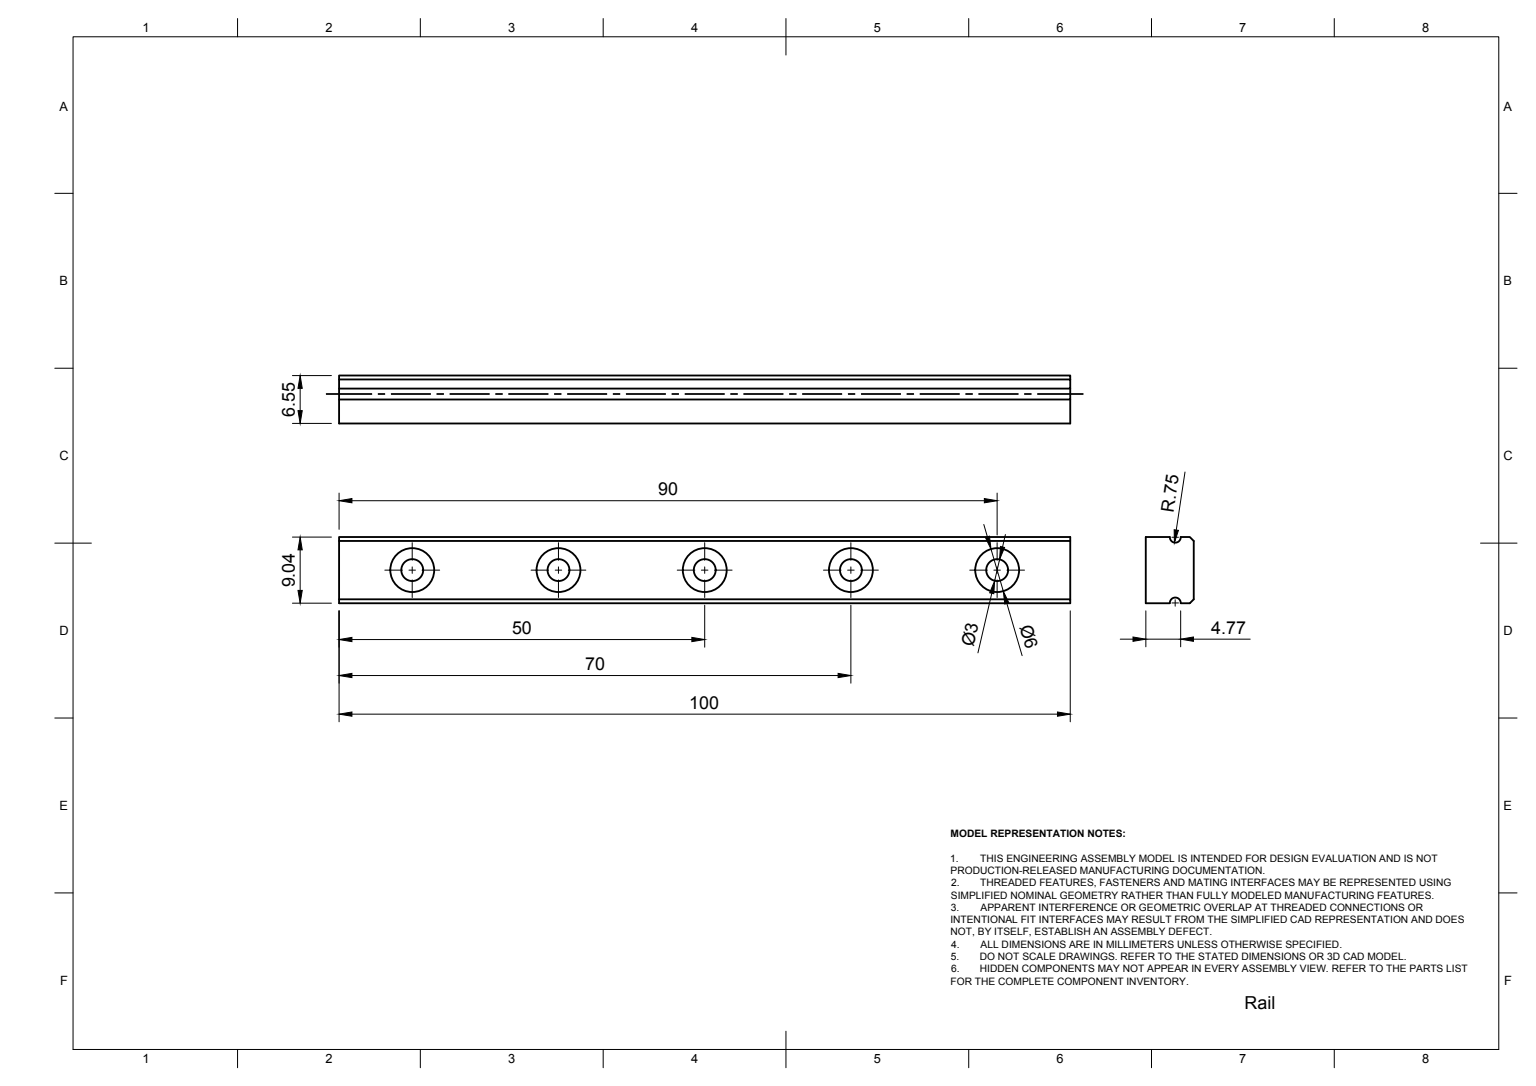
ISO-10303-21;
HEADER;
/* Generated by software containing ST-Developer
 * from STEP Tools, Inc. (www.steptools.com) 
 */

FILE_DESCRIPTION(
/* description */ (''),
/* implementation_level */ '2;1');

FILE_NAME(
/* name */ 'Rail.step',
/* time_stamp */ '2026-10-06T13:23:02-07:00',
/* author */ (''),
/* organization */ (''),
/* preprocessor_version */ 'ST-DEVELOPER v20.2',
/* originating_system */ 'Autodesk Translation Framework v15.15.0.0',
/* authorisation */ '');

FILE_SCHEMA (('AUTOMOTIVE_DESIGN { 1 0 10303 214 3 1 1 }'));
ENDSEC;

DATA;
#10=MECHANICAL_DESIGN_GEOMETRIC_PRESENTATION_REPRESENTATION('',(#75),#4994);
#55=SHAPE_REPRESENTATION_RELATIONSHIP('SRR','None',#5036,#65);
#65=ADVANCED_BREP_SHAPE_REPRESENTATION('',(#85),#4988);
#75=STYLED_ITEM('',(#5092),#85);
#85=MANIFOLD_SOLID_BREP('Body1',#2915);
#99=CYLINDRICAL_SURFACE('',#3150,1.5);
#100=CYLINDRICAL_SURFACE('',#3154,1.5);
#101=CYLINDRICAL_SURFACE('',#3158,1.5);
#102=CYLINDRICAL_SURFACE('',#3162,1.5);
#103=CYLINDRICAL_SURFACE('',#3166,1.5);
#104=CYLINDRICAL_SURFACE('',#3168,3.);
#105=CYLINDRICAL_SURFACE('',#3172,3.);
#106=CYLINDRICAL_SURFACE('',#3176,3.);
#107=CYLINDRICAL_SURFACE('',#3180,3.);
#108=CYLINDRICAL_SURFACE('',#3184,3.);
#109=CYLINDRICAL_SURFACE('',#3189,0.747295203682);
#110=CYLINDRICAL_SURFACE('',#3197,0.747295203682);
#131=FACE_BOUND('',#567,.T.);
#132=FACE_BOUND('',#568,.T.);
#133=FACE_BOUND('',#569,.T.);
#134=FACE_BOUND('',#570,.T.);
#135=FACE_BOUND('',#571,.T.);
#136=FACE_BOUND('',#583,.T.);
#137=FACE_BOUND('',#586,.T.);
#138=FACE_BOUND('',#589,.T.);
#139=FACE_BOUND('',#592,.T.);
#140=FACE_BOUND('',#595,.T.);
#141=FACE_BOUND('',#605,.T.);
#142=FACE_BOUND('',#606,.T.);
#143=FACE_BOUND('',#607,.T.);
#144=FACE_BOUND('',#608,.T.);
#145=FACE_BOUND('',#609,.T.);
#226=PLANE('',#3145);
#227=PLANE('',#3171);
#228=PLANE('',#3175);
#229=PLANE('',#3179);
#230=PLANE('',#3183);
#231=PLANE('',#3187);
#232=PLANE('',#3188);
#233=PLANE('',#3192);
#234=PLANE('',#3193);
#235=PLANE('',#3194);
#236=PLANE('',#3196);
#237=PLANE('',#3199);
#238=PLANE('',#3200);
#239=PLANE('',#3201);
#240=PLANE('',#3202);
#379=FACE_OUTER_BOUND('',#565,.T.);
#380=FACE_OUTER_BOUND('',#566,.T.);
#381=FACE_OUTER_BOUND('',#572,.T.);
#382=FACE_OUTER_BOUND('',#573,.T.);
#383=FACE_OUTER_BOUND('',#574,.T.);
#384=FACE_OUTER_BOUND('',#575,.T.);
#385=FACE_OUTER_BOUND('',#576,.T.);
#386=FACE_OUTER_BOUND('',#577,.T.);
#387=FACE_OUTER_BOUND('',#578,.T.);
#388=FACE_OUTER_BOUND('',#579,.T.);
#389=FACE_OUTER_BOUND('',#580,.T.);
#390=FACE_OUTER_BOUND('',#581,.T.);
#391=FACE_OUTER_BOUND('',#582,.T.);
#392=FACE_OUTER_BOUND('',#584,.T.);
#393=FACE_OUTER_BOUND('',#585,.T.);
#394=FACE_OUTER_BOUND('',#587,.T.);
#395=FACE_OUTER_BOUND('',#588,.T.);
#396=FACE_OUTER_BOUND('',#590,.T.);
#397=FACE_OUTER_BOUND('',#591,.T.);
#398=FACE_OUTER_BOUND('',#593,.T.);
#399=FACE_OUTER_BOUND('',#594,.T.);
#400=FACE_OUTER_BOUND('',#596,.T.);
#401=FACE_OUTER_BOUND('',#597,.T.);
#402=FACE_OUTER_BOUND('',#598,.T.);
#403=FACE_OUTER_BOUND('',#599,.T.);
#404=FACE_OUTER_BOUND('',#600,.T.);
#405=FACE_OUTER_BOUND('',#601,.T.);
#406=FACE_OUTER_BOUND('',#602,.T.);
#407=FACE_OUTER_BOUND('',#603,.T.);
#408=FACE_OUTER_BOUND('',#604,.T.);
#409=FACE_OUTER_BOUND('',#610,.T.);
#410=FACE_OUTER_BOUND('',#611,.T.);
#565=EDGE_LOOP('',(#2248,#2249,#2250,#2251));
#566=EDGE_LOOP('',(#2252,#2253,#2254,#2255));
#567=EDGE_LOOP('',(#2256));
#568=EDGE_LOOP('',(#2257));
#569=EDGE_LOOP('',(#2258));
#570=EDGE_LOOP('',(#2259));
#571=EDGE_LOOP('',(#2260));
#572=EDGE_LOOP('',(#2261,#2262,#2263,#2264));
#573=EDGE_LOOP('',(#2265,#2266,#2267,#2268));
#574=EDGE_LOOP('',(#2269,#2270,#2271,#2272));
#575=EDGE_LOOP('',(#2273,#2274,#2275,#2276));
#576=EDGE_LOOP('',(#2277,#2278,#2279,#2280));
#577=EDGE_LOOP('',(#2281,#2282,#2283,#2284));
#578=EDGE_LOOP('',(#2285,#2286,#2287,#2288));
#579=EDGE_LOOP('',(#2289,#2290,#2291,#2292));
#580=EDGE_LOOP('',(#2293,#2294,#2295,#2296));
#581=EDGE_LOOP('',(#2297,#2298,#2299,#2300));
#582=EDGE_LOOP('',(#2301));
#583=EDGE_LOOP('',(#2302));
#584=EDGE_LOOP('',(#2303,#2304,#2305,#2306));
#585=EDGE_LOOP('',(#2307));
#586=EDGE_LOOP('',(#2308));
#587=EDGE_LOOP('',(#2309,#2310,#2311,#2312));
#588=EDGE_LOOP('',(#2313));
#589=EDGE_LOOP('',(#2314));
#590=EDGE_LOOP('',(#2315,#2316,#2317,#2318));
#591=EDGE_LOOP('',(#2319));
#592=EDGE_LOOP('',(#2320));
#593=EDGE_LOOP('',(#2321,#2322,#2323,#2324));
#594=EDGE_LOOP('',(#2325));
#595=EDGE_LOOP('',(#2326));
#596=EDGE_LOOP('',(#2327,#2328,#2329,#2330));
#597=EDGE_LOOP('',(#2331,#2332,#2333,#2334));
#598=EDGE_LOOP('',(#2335,#2336,#2337,#2338));
#599=EDGE_LOOP('',(#2339,#2340,#2341,#2342));
#600=EDGE_LOOP('',(#2343,#2344,#2345,#2346,#2347,#2348,#2349,#2350,#2351,
#2352));
#601=EDGE_LOOP('',(#2353,#2354,#2355,#2356));
#602=EDGE_LOOP('',(#2357,#2358,#2359,#2360));
#603=EDGE_LOOP('',(#2361,#2362,#2363,#2364));
#604=EDGE_LOOP('',(#2365,#2366,#2367,#2368));
#605=EDGE_LOOP('',(#2369));
#606=EDGE_LOOP('',(#2370));
#607=EDGE_LOOP('',(#2371));
#608=EDGE_LOOP('',(#2372));
#609=EDGE_LOOP('',(#2373));
#610=EDGE_LOOP('',(#2374,#2375,#2376,#2377));
#611=EDGE_LOOP('',(#2378,#2379,#2380,#2381,#2382,#2383,#2384,#2385,#2386,
#2387));
#810=LINE('',#4463,#1103);
#811=LINE('',#4468,#1104);
#812=LINE('',#4470,#1105);
#813=LINE('',#4472,#1106);
#814=LINE('',#4473,#1107);
#815=LINE('',#4485,#1108);
#816=LINE('',#4489,#1109);
#817=LINE('',#4493,#1110);
#818=LINE('',#4497,#1111);
#819=LINE('',#4501,#1112);
#820=LINE('',#4505,#1113);
#821=LINE('',#4509,#1114);
#822=LINE('',#4513,#1115);
#823=LINE('',#4517,#1116);
#824=LINE('',#4522,#1117);
#825=LINE('',#4529,#1118);
#826=LINE('',#4536,#1119);
#827=LINE('',#4543,#1120);
#828=LINE('',#4550,#1121);
#829=LINE('',#4556,#1122);
#830=LINE('',#4558,#1123);
#831=LINE('',#4560,#1124);
#832=LINE('',#4561,#1125);
#833=LINE('',#4566,#1126);
#834=LINE('',#4569,#1127);
#835=LINE('',#4570,#1128);
#836=LINE('',#4574,#1129);
#837=LINE('',#4575,#1130);
#838=LINE('',#4576,#1131);
#839=LINE('',#4580,#1132);
#840=LINE('',#4582,#1133);
#841=LINE('',#4585,#1134);
#842=LINE('',#4586,#1135);
#843=LINE('',#4589,#1136);
#844=LINE('',#4591,#1137);
#845=LINE('',#4592,#1138);
#846=LINE('',#4596,#1139);
#847=LINE('',#4598,#1140);
#848=LINE('',#4601,#1141);
#849=LINE('',#4602,#1142);
#850=LINE('',#4604,#1143);
#1103=VECTOR('',#3644,1.75);
#1104=VECTOR('',#3649,10.);
#1105=VECTOR('',#3650,10.);
#1106=VECTOR('',#3651,10.);
#1107=VECTOR('',#3652,10.);
#1108=VECTOR('',#3665,1.5);
#1109=VECTOR('',#3670,1.75);
#1110=VECTOR('',#3675,1.5);
#1111=VECTOR('',#3680,1.75);
#1112=VECTOR('',#3685,1.5);
#1113=VECTOR('',#3690,1.75);
#1114=VECTOR('',#3695,1.5);
#1115=VECTOR('',#3700,1.75);
#1116=VECTOR('',#3705,1.5);
#1117=VECTOR('',#3710,3.);
#1118=VECTOR('',#3719,3.);
#1119=VECTOR('',#3728,3.);
#1120=VECTOR('',#3737,3.);
#1121=VECTOR('',#3746,3.);
#1122=VECTOR('',#3753,10.);
#1123=VECTOR('',#3754,10.);
#1124=VECTOR('',#3755,10.);
#1125=VECTOR('',#3756,10.);
#1126=VECTOR('',#3761,10.);
#1127=VECTOR('',#3766,10.);
#1128=VECTOR('',#3767,10.);
#1129=VECTOR('',#3770,10.);
#1130=VECTOR('',#3771,10.);
#1131=VECTOR('',#3772,10.);
#1132=VECTOR('',#3775,10.);
#1133=VECTOR('',#3776,10.);
#1134=VECTOR('',#3779,10.);
#1135=VECTOR('',#3780,10.);
#1136=VECTOR('',#3783,10.);
#1137=VECTOR('',#3784,10.);
#1138=VECTOR('',#3785,10.);
#1139=VECTOR('',#3790,10.);
#1140=VECTOR('',#3793,10.);
#1141=VECTOR('',#3796,10.);
#1142=VECTOR('',#3797,10.);
#1143=VECTOR('',#3800,10.);
#1316=CIRCLE('',#3143,1.5);
#1317=CIRCLE('',#3144,2.);
#1318=CIRCLE('',#3146,2.);
#1319=CIRCLE('',#3147,2.);
#1320=CIRCLE('',#3148,2.);
#1321=CIRCLE('',#3149,2.);
#1322=CIRCLE('',#3151,1.5);
#1323=CIRCLE('',#3153,1.5);
#1324=CIRCLE('',#3155,1.5);
#1325=CIRCLE('',#3157,1.5);
#1326=CIRCLE('',#3159,1.5);
#1327=CIRCLE('',#3161,1.5);
#1328=CIRCLE('',#3163,1.5);
#1329=CIRCLE('',#3165,1.5);
#1330=CIRCLE('',#3167,1.5);
#1331=CIRCLE('',#3169,3.);
#1332=CIRCLE('',#3170,3.);
#1333=CIRCLE('',#3173,3.);
#1334=CIRCLE('',#3174,3.);
#1335=CIRCLE('',#3177,3.);
#1336=CIRCLE('',#3178,3.);
#1337=CIRCLE('',#3181,3.);
#1338=CIRCLE('',#3182,3.);
#1339=CIRCLE('',#3185,3.);
#1340=CIRCLE('',#3186,3.);
#1341=CIRCLE('',#3190,0.747295203682);
#1342=CIRCLE('',#3191,0.747295203682);
#1343=CIRCLE('',#3195,0.747295203682);
#1344=CIRCLE('',#3198,0.747295203682);
#1445=VERTEX_POINT('',#4460);
#1446=VERTEX_POINT('',#4462);
#1447=VERTEX_POINT('',#4466);
#1448=VERTEX_POINT('',#4467);
#1449=VERTEX_POINT('',#4469);
#1450=VERTEX_POINT('',#4471);
#1451=VERTEX_POINT('',#4474);
#1452=VERTEX_POINT('',#4476);
#1453=VERTEX_POINT('',#4478);
#1454=VERTEX_POINT('',#4480);
#1455=VERTEX_POINT('',#4483);
#1456=VERTEX_POINT('',#4487);
#1457=VERTEX_POINT('',#4491);
#1458=VERTEX_POINT('',#4495);
#1459=VERTEX_POINT('',#4499);
#1460=VERTEX_POINT('',#4503);
#1461=VERTEX_POINT('',#4507);
#1462=VERTEX_POINT('',#4511);
#1463=VERTEX_POINT('',#4515);
#1464=VERTEX_POINT('',#4519);
#1465=VERTEX_POINT('',#4521);
#1466=VERTEX_POINT('',#4526);
#1467=VERTEX_POINT('',#4528);
#1468=VERTEX_POINT('',#4533);
#1469=VERTEX_POINT('',#4535);
#1470=VERTEX_POINT('',#4540);
#1471=VERTEX_POINT('',#4542);
#1472=VERTEX_POINT('',#4547);
#1473=VERTEX_POINT('',#4549);
#1474=VERTEX_POINT('',#4554);
#1475=VERTEX_POINT('',#4555);
#1476=VERTEX_POINT('',#4557);
#1477=VERTEX_POINT('',#4559);
#1478=VERTEX_POINT('',#4563);
#1479=VERTEX_POINT('',#4565);
#1480=VERTEX_POINT('',#4572);
#1481=VERTEX_POINT('',#4573);
#1482=VERTEX_POINT('',#4578);
#1483=VERTEX_POINT('',#4579);
#1484=VERTEX_POINT('',#4581);
#1485=VERTEX_POINT('',#4583);
#1486=VERTEX_POINT('',#4588);
#1487=VERTEX_POINT('',#4590);
#1488=VERTEX_POINT('',#4594);
#1489=VERTEX_POINT('',#4600);
#1738=EDGE_CURVE('',#1445,#1445,#1316,.T.);
#1739=EDGE_CURVE('',#1445,#1446,#810,.T.);
#1740=EDGE_CURVE('',#1446,#1446,#1317,.T.);
#1741=EDGE_CURVE('',#1447,#1448,#811,.T.);
#1742=EDGE_CURVE('',#1448,#1449,#812,.T.);
#1743=EDGE_CURVE('',#1450,#1449,#813,.T.);
#1744=EDGE_CURVE('',#1447,#1450,#814,.T.);
#1745=EDGE_CURVE('',#1451,#1451,#1318,.T.);
#1746=EDGE_CURVE('',#1452,#1452,#1319,.T.);
#1747=EDGE_CURVE('',#1453,#1453,#1320,.T.);
#1748=EDGE_CURVE('',#1454,#1454,#1321,.T.);
#1749=EDGE_CURVE('',#1455,#1455,#1322,.T.);
#1750=EDGE_CURVE('',#1455,#1445,#815,.T.);
#1751=EDGE_CURVE('',#1456,#1456,#1323,.T.);
#1752=EDGE_CURVE('',#1456,#1451,#816,.T.);
#1753=EDGE_CURVE('',#1457,#1457,#1324,.T.);
#1754=EDGE_CURVE('',#1457,#1456,#817,.T.);
#1755=EDGE_CURVE('',#1458,#1458,#1325,.T.);
#1756=EDGE_CURVE('',#1458,#1454,#818,.T.);
#1757=EDGE_CURVE('',#1459,#1459,#1326,.T.);
#1758=EDGE_CURVE('',#1459,#1458,#819,.T.);
#1759=EDGE_CURVE('',#1460,#1460,#1327,.T.);
#1760=EDGE_CURVE('',#1460,#1452,#820,.T.);
#1761=EDGE_CURVE('',#1461,#1461,#1328,.T.);
#1762=EDGE_CURVE('',#1461,#1460,#821,.T.);
#1763=EDGE_CURVE('',#1462,#1462,#1329,.T.);
#1764=EDGE_CURVE('',#1462,#1453,#822,.T.);
#1765=EDGE_CURVE('',#1463,#1463,#1330,.T.);
#1766=EDGE_CURVE('',#1463,#1462,#823,.T.);
#1767=EDGE_CURVE('',#1464,#1464,#1331,.T.);
#1768=EDGE_CURVE('',#1464,#1465,#824,.T.);
#1769=EDGE_CURVE('',#1465,#1465,#1332,.T.);
#1770=EDGE_CURVE('',#1466,#1466,#1333,.T.);
#1771=EDGE_CURVE('',#1466,#1467,#825,.T.);
#1772=EDGE_CURVE('',#1467,#1467,#1334,.T.);
#1773=EDGE_CURVE('',#1468,#1468,#1335,.T.);
#1774=EDGE_CURVE('',#1468,#1469,#826,.T.);
#1775=EDGE_CURVE('',#1469,#1469,#1336,.T.);
#1776=EDGE_CURVE('',#1470,#1470,#1337,.T.);
#1777=EDGE_CURVE('',#1470,#1471,#827,.T.);
#1778=EDGE_CURVE('',#1471,#1471,#1338,.T.);
#1779=EDGE_CURVE('',#1472,#1472,#1339,.T.);
#1780=EDGE_CURVE('',#1472,#1473,#828,.T.);
#1781=EDGE_CURVE('',#1473,#1473,#1340,.T.);
#1782=EDGE_CURVE('',#1474,#1475,#829,.T.);
#1783=EDGE_CURVE('',#1475,#1476,#830,.T.);
#1784=EDGE_CURVE('',#1476,#1477,#831,.T.);
#1785=EDGE_CURVE('',#1477,#1474,#832,.T.);
#1786=EDGE_CURVE('',#1476,#1478,#1341,.T.);
#1787=EDGE_CURVE('',#1478,#1479,#833,.T.);
#1788=EDGE_CURVE('',#1479,#1477,#1342,.T.);
#1789=EDGE_CURVE('',#1478,#1450,#834,.T.);
#1790=EDGE_CURVE('',#1449,#1479,#835,.T.);
#1791=EDGE_CURVE('',#1480,#1481,#836,.T.);
#1792=EDGE_CURVE('',#1480,#1475,#837,.T.);
#1793=EDGE_CURVE('',#1474,#1481,#838,.T.);
#1794=EDGE_CURVE('',#1482,#1483,#839,.T.);
#1795=EDGE_CURVE('',#1483,#1484,#840,.T.);
#1796=EDGE_CURVE('',#1484,#1485,#1343,.T.);
#1797=EDGE_CURVE('',#1485,#1447,#841,.T.);
#1798=EDGE_CURVE('',#1482,#1480,#842,.T.);
#1799=EDGE_CURVE('',#1486,#1483,#843,.T.);
#1800=EDGE_CURVE('',#1487,#1486,#844,.T.);
#1801=EDGE_CURVE('',#1484,#1487,#845,.T.);
#1802=EDGE_CURVE('',#1488,#1487,#1344,.T.);
#1803=EDGE_CURVE('',#1485,#1488,#846,.T.);
#1804=EDGE_CURVE('',#1448,#1488,#847,.T.);
#1805=EDGE_CURVE('',#1489,#1481,#848,.T.);
#1806=EDGE_CURVE('',#1482,#1489,#849,.T.);
#1807=EDGE_CURVE('',#1486,#1489,#850,.T.);
#2248=ORIENTED_EDGE('',*,*,#1738,.T.);
#2249=ORIENTED_EDGE('',*,*,#1739,.T.);
#2250=ORIENTED_EDGE('',*,*,#1740,.T.);
#2251=ORIENTED_EDGE('',*,*,#1739,.F.);
#2252=ORIENTED_EDGE('',*,*,#1741,.T.);
#2253=ORIENTED_EDGE('',*,*,#1742,.T.);
#2254=ORIENTED_EDGE('',*,*,#1743,.F.);
#2255=ORIENTED_EDGE('',*,*,#1744,.F.);
#2256=ORIENTED_EDGE('',*,*,#1745,.F.);
#2257=ORIENTED_EDGE('',*,*,#1746,.F.);
#2258=ORIENTED_EDGE('',*,*,#1747,.F.);
#2259=ORIENTED_EDGE('',*,*,#1748,.F.);
#2260=ORIENTED_EDGE('',*,*,#1740,.F.);
#2261=ORIENTED_EDGE('',*,*,#1749,.T.);
#2262=ORIENTED_EDGE('',*,*,#1750,.T.);
#2263=ORIENTED_EDGE('',*,*,#1738,.F.);
#2264=ORIENTED_EDGE('',*,*,#1750,.F.);
#2265=ORIENTED_EDGE('',*,*,#1751,.T.);
#2266=ORIENTED_EDGE('',*,*,#1752,.T.);
#2267=ORIENTED_EDGE('',*,*,#1745,.T.);
#2268=ORIENTED_EDGE('',*,*,#1752,.F.);
#2269=ORIENTED_EDGE('',*,*,#1753,.T.);
#2270=ORIENTED_EDGE('',*,*,#1754,.T.);
#2271=ORIENTED_EDGE('',*,*,#1751,.F.);
#2272=ORIENTED_EDGE('',*,*,#1754,.F.);
#2273=ORIENTED_EDGE('',*,*,#1755,.T.);
#2274=ORIENTED_EDGE('',*,*,#1756,.T.);
#2275=ORIENTED_EDGE('',*,*,#1748,.T.);
#2276=ORIENTED_EDGE('',*,*,#1756,.F.);
#2277=ORIENTED_EDGE('',*,*,#1757,.T.);
#2278=ORIENTED_EDGE('',*,*,#1758,.T.);
#2279=ORIENTED_EDGE('',*,*,#1755,.F.);
#2280=ORIENTED_EDGE('',*,*,#1758,.F.);
#2281=ORIENTED_EDGE('',*,*,#1759,.T.);
#2282=ORIENTED_EDGE('',*,*,#1760,.T.);
#2283=ORIENTED_EDGE('',*,*,#1746,.T.);
#2284=ORIENTED_EDGE('',*,*,#1760,.F.);
#2285=ORIENTED_EDGE('',*,*,#1761,.T.);
#2286=ORIENTED_EDGE('',*,*,#1762,.T.);
#2287=ORIENTED_EDGE('',*,*,#1759,.F.);
#2288=ORIENTED_EDGE('',*,*,#1762,.F.);
#2289=ORIENTED_EDGE('',*,*,#1763,.T.);
#2290=ORIENTED_EDGE('',*,*,#1764,.T.);
#2291=ORIENTED_EDGE('',*,*,#1747,.T.);
#2292=ORIENTED_EDGE('',*,*,#1764,.F.);
#2293=ORIENTED_EDGE('',*,*,#1765,.T.);
#2294=ORIENTED_EDGE('',*,*,#1766,.T.);
#2295=ORIENTED_EDGE('',*,*,#1763,.F.);
#2296=ORIENTED_EDGE('',*,*,#1766,.F.);
#2297=ORIENTED_EDGE('',*,*,#1767,.F.);
#2298=ORIENTED_EDGE('',*,*,#1768,.T.);
#2299=ORIENTED_EDGE('',*,*,#1769,.T.);
#2300=ORIENTED_EDGE('',*,*,#1768,.F.);
#2301=ORIENTED_EDGE('',*,*,#1769,.F.);
#2302=ORIENTED_EDGE('',*,*,#1757,.F.);
#2303=ORIENTED_EDGE('',*,*,#1770,.F.);
#2304=ORIENTED_EDGE('',*,*,#1771,.T.);
#2305=ORIENTED_EDGE('',*,*,#1772,.T.);
#2306=ORIENTED_EDGE('',*,*,#1771,.F.);
#2307=ORIENTED_EDGE('',*,*,#1772,.F.);
#2308=ORIENTED_EDGE('',*,*,#1761,.F.);
#2309=ORIENTED_EDGE('',*,*,#1773,.F.);
#2310=ORIENTED_EDGE('',*,*,#1774,.T.);
#2311=ORIENTED_EDGE('',*,*,#1775,.T.);
#2312=ORIENTED_EDGE('',*,*,#1774,.F.);
#2313=ORIENTED_EDGE('',*,*,#1775,.F.);
#2314=ORIENTED_EDGE('',*,*,#1753,.F.);
#2315=ORIENTED_EDGE('',*,*,#1776,.F.);
#2316=ORIENTED_EDGE('',*,*,#1777,.T.);
#2317=ORIENTED_EDGE('',*,*,#1778,.T.);
#2318=ORIENTED_EDGE('',*,*,#1777,.F.);
#2319=ORIENTED_EDGE('',*,*,#1778,.F.);
#2320=ORIENTED_EDGE('',*,*,#1765,.F.);
#2321=ORIENTED_EDGE('',*,*,#1779,.F.);
#2322=ORIENTED_EDGE('',*,*,#1780,.T.);
#2323=ORIENTED_EDGE('',*,*,#1781,.T.);
#2324=ORIENTED_EDGE('',*,*,#1780,.F.);
#2325=ORIENTED_EDGE('',*,*,#1781,.F.);
#2326=ORIENTED_EDGE('',*,*,#1749,.F.);
#2327=ORIENTED_EDGE('',*,*,#1782,.T.);
#2328=ORIENTED_EDGE('',*,*,#1783,.T.);
#2329=ORIENTED_EDGE('',*,*,#1784,.T.);
#2330=ORIENTED_EDGE('',*,*,#1785,.T.);
#2331=ORIENTED_EDGE('',*,*,#1784,.F.);
#2332=ORIENTED_EDGE('',*,*,#1786,.T.);
#2333=ORIENTED_EDGE('',*,*,#1787,.T.);
#2334=ORIENTED_EDGE('',*,*,#1788,.T.);
#2335=ORIENTED_EDGE('',*,*,#1787,.F.);
#2336=ORIENTED_EDGE('',*,*,#1789,.T.);
#2337=ORIENTED_EDGE('',*,*,#1743,.T.);
#2338=ORIENTED_EDGE('',*,*,#1790,.T.);
#2339=ORIENTED_EDGE('',*,*,#1791,.F.);
#2340=ORIENTED_EDGE('',*,*,#1792,.T.);
#2341=ORIENTED_EDGE('',*,*,#1782,.F.);
#2342=ORIENTED_EDGE('',*,*,#1793,.T.);
#2343=ORIENTED_EDGE('',*,*,#1794,.T.);
#2344=ORIENTED_EDGE('',*,*,#1795,.T.);
#2345=ORIENTED_EDGE('',*,*,#1796,.T.);
#2346=ORIENTED_EDGE('',*,*,#1797,.T.);
#2347=ORIENTED_EDGE('',*,*,#1744,.T.);
#2348=ORIENTED_EDGE('',*,*,#1789,.F.);
#2349=ORIENTED_EDGE('',*,*,#1786,.F.);
#2350=ORIENTED_EDGE('',*,*,#1783,.F.);
#2351=ORIENTED_EDGE('',*,*,#1792,.F.);
#2352=ORIENTED_EDGE('',*,*,#1798,.F.);
#2353=ORIENTED_EDGE('',*,*,#1799,.F.);
#2354=ORIENTED_EDGE('',*,*,#1800,.F.);
#2355=ORIENTED_EDGE('',*,*,#1801,.F.);
#2356=ORIENTED_EDGE('',*,*,#1795,.F.);
#2357=ORIENTED_EDGE('',*,*,#1801,.T.);
#2358=ORIENTED_EDGE('',*,*,#1802,.F.);
#2359=ORIENTED_EDGE('',*,*,#1803,.F.);
#2360=ORIENTED_EDGE('',*,*,#1796,.F.);
#2361=ORIENTED_EDGE('',*,*,#1803,.T.);
#2362=ORIENTED_EDGE('',*,*,#1804,.F.);
#2363=ORIENTED_EDGE('',*,*,#1741,.F.);
#2364=ORIENTED_EDGE('',*,*,#1797,.F.);
#2365=ORIENTED_EDGE('',*,*,#1805,.F.);
#2366=ORIENTED_EDGE('',*,*,#1806,.F.);
#2367=ORIENTED_EDGE('',*,*,#1798,.T.);
#2368=ORIENTED_EDGE('',*,*,#1791,.T.);
#2369=ORIENTED_EDGE('',*,*,#1779,.T.);
#2370=ORIENTED_EDGE('',*,*,#1776,.T.);
#2371=ORIENTED_EDGE('',*,*,#1773,.T.);
#2372=ORIENTED_EDGE('',*,*,#1770,.T.);
#2373=ORIENTED_EDGE('',*,*,#1767,.T.);
#2374=ORIENTED_EDGE('',*,*,#1806,.T.);
#2375=ORIENTED_EDGE('',*,*,#1807,.F.);
#2376=ORIENTED_EDGE('',*,*,#1799,.T.);
#2377=ORIENTED_EDGE('',*,*,#1794,.F.);
#2378=ORIENTED_EDGE('',*,*,#1807,.T.);
#2379=ORIENTED_EDGE('',*,*,#1805,.T.);
#2380=ORIENTED_EDGE('',*,*,#1793,.F.);
#2381=ORIENTED_EDGE('',*,*,#1785,.F.);
#2382=ORIENTED_EDGE('',*,*,#1788,.F.);
#2383=ORIENTED_EDGE('',*,*,#1790,.F.);
#2384=ORIENTED_EDGE('',*,*,#1742,.F.);
#2385=ORIENTED_EDGE('',*,*,#1804,.T.);
#2386=ORIENTED_EDGE('',*,*,#1802,.T.);
#2387=ORIENTED_EDGE('',*,*,#1800,.T.);
#2728=CONICAL_SURFACE('',#3142,1.75,0.785398163397447);
#2729=CONICAL_SURFACE('',#3152,1.75,0.785398163397447);
#2730=CONICAL_SURFACE('',#3156,1.75,0.785398163397449);
#2731=CONICAL_SURFACE('',#3160,1.75,0.78539816339745);
#2732=CONICAL_SURFACE('',#3164,1.75,0.785398163397447);
#2809=ADVANCED_FACE('',(#379),#2728,.F.);
#2810=ADVANCED_FACE('',(#380,#131,#132,#133,#134,#135),#226,.T.);
#2811=ADVANCED_FACE('',(#381),#99,.F.);
#2812=ADVANCED_FACE('',(#382),#2729,.F.);
#2813=ADVANCED_FACE('',(#383),#100,.F.);
#2814=ADVANCED_FACE('',(#384),#2730,.F.);
#2815=ADVANCED_FACE('',(#385),#101,.F.);
#2816=ADVANCED_FACE('',(#386),#2731,.F.);
#2817=ADVANCED_FACE('',(#387),#102,.F.);
#2818=ADVANCED_FACE('',(#388),#2732,.F.);
#2819=ADVANCED_FACE('',(#389),#103,.F.);
#2820=ADVANCED_FACE('',(#390),#104,.F.);
#2821=ADVANCED_FACE('',(#391,#136),#227,.T.);
#2822=ADVANCED_FACE('',(#392),#105,.F.);
#2823=ADVANCED_FACE('',(#393,#137),#228,.T.);
#2824=ADVANCED_FACE('',(#394),#106,.F.);
#2825=ADVANCED_FACE('',(#395,#138),#229,.T.);
#2826=ADVANCED_FACE('',(#396),#107,.F.);
#2827=ADVANCED_FACE('',(#397,#139),#230,.T.);
#2828=ADVANCED_FACE('',(#398),#108,.F.);
#2829=ADVANCED_FACE('',(#399,#140),#231,.T.);
#2830=ADVANCED_FACE('',(#400),#232,.F.);
#2831=ADVANCED_FACE('',(#401),#109,.F.);
#2832=ADVANCED_FACE('',(#402),#233,.F.);
#2833=ADVANCED_FACE('',(#403),#234,.F.);
#2834=ADVANCED_FACE('',(#404),#235,.F.);
#2835=ADVANCED_FACE('',(#405),#236,.T.);
#2836=ADVANCED_FACE('',(#406),#110,.F.);
#2837=ADVANCED_FACE('',(#407),#237,.T.);
#2838=ADVANCED_FACE('',(#408,#141,#142,#143,#144,#145),#238,.T.);
#2839=ADVANCED_FACE('',(#409),#239,.T.);
#2840=ADVANCED_FACE('',(#410),#240,.T.);
#2915=CLOSED_SHELL('',(#2809,#2810,#2811,#2812,#2813,#2814,#2815,#2816,
#2817,#2818,#2819,#2820,#2821,#2822,#2823,#2824,#2825,#2826,#2827,#2828,
#2829,#2830,#2831,#2832,#2833,#2834,#2835,#2836,#2837,#2838,#2839,#2840));
#3141=AXIS2_PLACEMENT_3D('',#4458,#3638,#3639);
#3142=AXIS2_PLACEMENT_3D('',#4459,#3640,#3641);
#3143=AXIS2_PLACEMENT_3D('',#4461,#3642,#3643);
#3144=AXIS2_PLACEMENT_3D('',#4464,#3645,#3646);
#3145=AXIS2_PLACEMENT_3D('',#4465,#3647,#3648);
#3146=AXIS2_PLACEMENT_3D('',#4475,#3653,#3654);
#3147=AXIS2_PLACEMENT_3D('',#4477,#3655,#3656);
#3148=AXIS2_PLACEMENT_3D('',#4479,#3657,#3658);
#3149=AXIS2_PLACEMENT_3D('',#4481,#3659,#3660);
#3150=AXIS2_PLACEMENT_3D('',#4482,#3661,#3662);
#3151=AXIS2_PLACEMENT_3D('',#4484,#3663,#3664);
#3152=AXIS2_PLACEMENT_3D('',#4486,#3666,#3667);
#3153=AXIS2_PLACEMENT_3D('',#4488,#3668,#3669);
#3154=AXIS2_PLACEMENT_3D('',#4490,#3671,#3672);
#3155=AXIS2_PLACEMENT_3D('',#4492,#3673,#3674);
#3156=AXIS2_PLACEMENT_3D('',#4494,#3676,#3677);
#3157=AXIS2_PLACEMENT_3D('',#4496,#3678,#3679);
#3158=AXIS2_PLACEMENT_3D('',#4498,#3681,#3682);
#3159=AXIS2_PLACEMENT_3D('',#4500,#3683,#3684);
#3160=AXIS2_PLACEMENT_3D('',#4502,#3686,#3687);
#3161=AXIS2_PLACEMENT_3D('',#4504,#3688,#3689);
#3162=AXIS2_PLACEMENT_3D('',#4506,#3691,#3692);
#3163=AXIS2_PLACEMENT_3D('',#4508,#3693,#3694);
#3164=AXIS2_PLACEMENT_3D('',#4510,#3696,#3697);
#3165=AXIS2_PLACEMENT_3D('',#4512,#3698,#3699);
#3166=AXIS2_PLACEMENT_3D('',#4514,#3701,#3702);
#3167=AXIS2_PLACEMENT_3D('',#4516,#3703,#3704);
#3168=AXIS2_PLACEMENT_3D('',#4518,#3706,#3707);
#3169=AXIS2_PLACEMENT_3D('',#4520,#3708,#3709);
#3170=AXIS2_PLACEMENT_3D('',#4523,#3711,#3712);
#3171=AXIS2_PLACEMENT_3D('',#4524,#3713,#3714);
#3172=AXIS2_PLACEMENT_3D('',#4525,#3715,#3716);
#3173=AXIS2_PLACEMENT_3D('',#4527,#3717,#3718);
#3174=AXIS2_PLACEMENT_3D('',#4530,#3720,#3721);
#3175=AXIS2_PLACEMENT_3D('',#4531,#3722,#3723);
#3176=AXIS2_PLACEMENT_3D('',#4532,#3724,#3725);
#3177=AXIS2_PLACEMENT_3D('',#4534,#3726,#3727);
#3178=AXIS2_PLACEMENT_3D('',#4537,#3729,#3730);
#3179=AXIS2_PLACEMENT_3D('',#4538,#3731,#3732);
#3180=AXIS2_PLACEMENT_3D('',#4539,#3733,#3734);
#3181=AXIS2_PLACEMENT_3D('',#4541,#3735,#3736);
#3182=AXIS2_PLACEMENT_3D('',#4544,#3738,#3739);
#3183=AXIS2_PLACEMENT_3D('',#4545,#3740,#3741);
#3184=AXIS2_PLACEMENT_3D('',#4546,#3742,#3743);
#3185=AXIS2_PLACEMENT_3D('',#4548,#3744,#3745);
#3186=AXIS2_PLACEMENT_3D('',#4551,#3747,#3748);
#3187=AXIS2_PLACEMENT_3D('',#4552,#3749,#3750);
#3188=AXIS2_PLACEMENT_3D('',#4553,#3751,#3752);
#3189=AXIS2_PLACEMENT_3D('',#4562,#3757,#3758);
#3190=AXIS2_PLACEMENT_3D('',#4564,#3759,#3760);
#3191=AXIS2_PLACEMENT_3D('',#4567,#3762,#3763);
#3192=AXIS2_PLACEMENT_3D('',#4568,#3764,#3765);
#3193=AXIS2_PLACEMENT_3D('',#4571,#3768,#3769);
#3194=AXIS2_PLACEMENT_3D('',#4577,#3773,#3774);
#3195=AXIS2_PLACEMENT_3D('',#4584,#3777,#3778);
#3196=AXIS2_PLACEMENT_3D('',#4587,#3781,#3782);
#3197=AXIS2_PLACEMENT_3D('',#4593,#3786,#3787);
#3198=AXIS2_PLACEMENT_3D('',#4595,#3788,#3789);
#3199=AXIS2_PLACEMENT_3D('',#4597,#3791,#3792);
#3200=AXIS2_PLACEMENT_3D('',#4599,#3794,#3795);
#3201=AXIS2_PLACEMENT_3D('',#4603,#3798,#3799);
#3202=AXIS2_PLACEMENT_3D('',#4605,#3801,#3802);
#3638=DIRECTION('axis',(0.,0.,1.));
#3639=DIRECTION('refdir',(1.,0.,0.));
#3640=DIRECTION('center_axis',(0.,0.,-1.));
#3641=DIRECTION('ref_axis',(-1.,0.,0.));
#3642=DIRECTION('center_axis',(0.,0.,1.));
#3643=DIRECTION('ref_axis',(-1.,0.,0.));
#3644=DIRECTION('',(0.707106781186547,-8.65956056235492E-17,-0.707106781186548));
#3645=DIRECTION('center_axis',(0.,0.,-1.));
#3646=DIRECTION('ref_axis',(-1.,0.,0.));
#3647=DIRECTION('center_axis',(0.,0.,-1.));
#3648=DIRECTION('ref_axis',(0.,1.,0.));
#3649=DIRECTION('',(1.,0.,0.));
#3650=DIRECTION('',(0.,-1.,0.));
#3651=DIRECTION('',(1.,0.,0.));
#3652=DIRECTION('',(0.,-1.,0.));
#3653=DIRECTION('center_axis',(0.,0.,-1.));
#3654=DIRECTION('ref_axis',(-1.,0.,0.));
#3655=DIRECTION('center_axis',(0.,0.,-1.));
#3656=DIRECTION('ref_axis',(-1.,0.,0.));
#3657=DIRECTION('center_axis',(0.,0.,-1.));
#3658=DIRECTION('ref_axis',(-1.,0.,0.));
#3659=DIRECTION('center_axis',(0.,0.,-1.));
#3660=DIRECTION('ref_axis',(-1.,0.,0.));
#3661=DIRECTION('center_axis',(0.,0.,-1.));
#3662=DIRECTION('ref_axis',(-1.,0.,0.));
#3663=DIRECTION('center_axis',(0.,0.,1.));
#3664=DIRECTION('ref_axis',(-1.,0.,0.));
#3665=DIRECTION('',(0.,0.,-1.));
#3666=DIRECTION('center_axis',(0.,0.,-1.));
#3667=DIRECTION('ref_axis',(-1.,0.,0.));
#3668=DIRECTION('center_axis',(0.,0.,1.));
#3669=DIRECTION('ref_axis',(-1.,0.,0.));
#3670=DIRECTION('',(0.707106781186547,-8.65956056235492E-17,-0.707106781186548));
#3671=DIRECTION('center_axis',(0.,0.,-1.));
#3672=DIRECTION('ref_axis',(-1.,0.,0.));
#3673=DIRECTION('center_axis',(0.,0.,1.));
#3674=DIRECTION('ref_axis',(-1.,0.,0.));
#3675=DIRECTION('',(0.,0.,-1.));
#3676=DIRECTION('center_axis',(0.,0.,-1.));
#3677=DIRECTION('ref_axis',(-1.,0.,0.));
#3678=DIRECTION('center_axis',(0.,0.,1.));
#3679=DIRECTION('ref_axis',(-1.,0.,0.));
#3680=DIRECTION('',(0.707106781186548,-8.65956056235494E-17,-0.707106781186547));
#3681=DIRECTION('center_axis',(0.,0.,-1.));
#3682=DIRECTION('ref_axis',(-1.,0.,0.));
#3683=DIRECTION('center_axis',(0.,0.,1.));
#3684=DIRECTION('ref_axis',(-1.,0.,0.));
#3685=DIRECTION('',(0.,0.,-1.));
#3686=DIRECTION('center_axis',(0.,0.,-1.));
#3687=DIRECTION('ref_axis',(-1.,0.,0.));
#3688=DIRECTION('center_axis',(0.,0.,1.));
#3689=DIRECTION('ref_axis',(-1.,0.,0.));
#3690=DIRECTION('',(0.707106781186549,-8.65956056235495E-17,-0.707106781186546));
#3691=DIRECTION('center_axis',(0.,0.,-1.));
#3692=DIRECTION('ref_axis',(-1.,0.,0.));
#3693=DIRECTION('center_axis',(0.,0.,1.));
#3694=DIRECTION('ref_axis',(-1.,0.,0.));
#3695=DIRECTION('',(0.,0.,-1.));
#3696=DIRECTION('center_axis',(0.,0.,-1.));
#3697=DIRECTION('ref_axis',(-1.,0.,0.));
#3698=DIRECTION('center_axis',(0.,0.,1.));
#3699=DIRECTION('ref_axis',(-1.,0.,0.));
#3700=DIRECTION('',(0.707106781186547,-8.65956056235492E-17,-0.707106781186548));
#3701=DIRECTION('center_axis',(0.,0.,-1.));
#3702=DIRECTION('ref_axis',(-1.,0.,0.));
#3703=DIRECTION('center_axis',(0.,0.,1.));
#3704=DIRECTION('ref_axis',(-1.,0.,0.));
#3705=DIRECTION('',(0.,0.,-1.));
#3706=DIRECTION('center_axis',(0.,0.,-1.));
#3707=DIRECTION('ref_axis',(-1.,0.,0.));
#3708=DIRECTION('center_axis',(0.,0.,-1.));
#3709=DIRECTION('ref_axis',(-1.,0.,0.));
#3710=DIRECTION('',(0.,0.,-1.));
#3711=DIRECTION('center_axis',(0.,0.,-1.));
#3712=DIRECTION('ref_axis',(-1.,0.,0.));
#3713=DIRECTION('center_axis',(0.,0.,1.));
#3714=DIRECTION('ref_axis',(-1.,0.,0.));
#3715=DIRECTION('center_axis',(0.,0.,-1.));
#3716=DIRECTION('ref_axis',(-1.,0.,0.));
#3717=DIRECTION('center_axis',(0.,0.,-1.));
#3718=DIRECTION('ref_axis',(-1.,0.,0.));
#3719=DIRECTION('',(0.,0.,-1.));
#3720=DIRECTION('center_axis',(0.,0.,-1.));
#3721=DIRECTION('ref_axis',(-1.,0.,0.));
#3722=DIRECTION('center_axis',(0.,0.,1.));
#3723=DIRECTION('ref_axis',(-1.,0.,0.));
#3724=DIRECTION('center_axis',(0.,0.,-1.));
#3725=DIRECTION('ref_axis',(-1.,0.,0.));
#3726=DIRECTION('center_axis',(0.,0.,-1.));
#3727=DIRECTION('ref_axis',(-1.,0.,0.));
#3728=DIRECTION('',(0.,0.,-1.));
#3729=DIRECTION('center_axis',(0.,0.,-1.));
#3730=DIRECTION('ref_axis',(-1.,0.,0.));
#3731=DIRECTION('center_axis',(0.,0.,1.));
#3732=DIRECTION('ref_axis',(-1.,0.,0.));
#3733=DIRECTION('center_axis',(0.,0.,-1.));
#3734=DIRECTION('ref_axis',(-1.,0.,0.));
#3735=DIRECTION('center_axis',(0.,0.,-1.));
#3736=DIRECTION('ref_axis',(-1.,0.,0.));
#3737=DIRECTION('',(0.,0.,-1.));
#3738=DIRECTION('center_axis',(0.,0.,-1.));
#3739=DIRECTION('ref_axis',(-1.,0.,0.));
#3740=DIRECTION('center_axis',(0.,0.,1.));
#3741=DIRECTION('ref_axis',(-1.,0.,0.));
#3742=DIRECTION('center_axis',(0.,0.,-1.));
#3743=DIRECTION('ref_axis',(-1.,0.,0.));
#3744=DIRECTION('center_axis',(0.,0.,-1.));
#3745=DIRECTION('ref_axis',(-1.,0.,0.));
#3746=DIRECTION('',(0.,0.,-1.));
#3747=DIRECTION('center_axis',(0.,0.,-1.));
#3748=DIRECTION('ref_axis',(-1.,0.,0.));
#3749=DIRECTION('center_axis',(0.,0.,1.));
#3750=DIRECTION('ref_axis',(-1.,0.,0.));
#3751=DIRECTION('center_axis',(0.,1.,0.));
#3752=DIRECTION('ref_axis',(0.,0.,1.));
#3753=DIRECTION('',(-1.,0.,0.));
#3754=DIRECTION('',(0.,0.,-1.));
#3755=DIRECTION('',(1.,0.,0.));
#3756=DIRECTION('',(0.,0.,1.));
#3757=DIRECTION('center_axis',(-1.,0.,0.));
#3758=DIRECTION('ref_axis',(0.,1.,1.18388150812306E-15));
#3759=DIRECTION('center_axis',(-1.,0.,0.));
#3760=DIRECTION('ref_axis',(0.,-0.0407335971034729,0.999170042618879));
#3761=DIRECTION('',(1.,0.,0.));
#3762=DIRECTION('center_axis',(1.,0.,0.));
#3763=DIRECTION('ref_axis',(0.,-0.0407335971034729,0.999170042618879));
#3764=DIRECTION('center_axis',(0.,1.,0.));
#3765=DIRECTION('ref_axis',(0.,0.,1.));
#3766=DIRECTION('',(0.,0.,-1.));
#3767=DIRECTION('',(0.,0.,1.));
#3768=DIRECTION('center_axis',(0.,0.706957380091336,-0.707256150722208));
#3769=DIRECTION('ref_axis',(0.,0.707256150722208,0.706957380091336));
#3770=DIRECTION('',(1.,0.,0.));
#3771=DIRECTION('',(0.,-0.707256150722208,-0.706957380091336));
#3772=DIRECTION('',(0.,0.707256150722208,0.706957380091336));
#3773=DIRECTION('center_axis',(1.,0.,0.));
#3774=DIRECTION('ref_axis',(0.,1.,0.));
#3775=DIRECTION('',(0.,0.707256150722208,-0.706957380091336));
#3776=DIRECTION('',(0.,0.,-1.));
#3777=DIRECTION('center_axis',(1.,0.,0.));
#3778=DIRECTION('ref_axis',(0.,0.0407335971034729,0.999170042618879));
#3779=DIRECTION('',(0.,0.,-1.));
#3780=DIRECTION('',(0.,-1.,0.));
#3781=DIRECTION('center_axis',(0.,1.,0.));
#3782=DIRECTION('ref_axis',(0.,0.,1.));
#3783=DIRECTION('',(-1.,0.,0.));
#3784=DIRECTION('',(0.,0.,1.));
#3785=DIRECTION('',(1.,0.,0.));
#3786=DIRECTION('center_axis',(1.,0.,0.));
#3787=DIRECTION('ref_axis',(0.,-1.,1.18388150812306E-15));
#3788=DIRECTION('center_axis',(-1.,0.,0.));
#3789=DIRECTION('ref_axis',(0.,0.0407335971034729,0.999170042618879));
#3790=DIRECTION('',(1.,0.,0.));
#3791=DIRECTION('center_axis',(0.,1.,0.));
#3792=DIRECTION('ref_axis',(0.,0.,1.));
#3793=DIRECTION('',(0.,0.,1.));
#3794=DIRECTION('center_axis',(0.,0.,1.));
#3795=DIRECTION('ref_axis',(0.,-1.,0.));
#3796=DIRECTION('',(0.,-1.,0.));
#3797=DIRECTION('',(1.,0.,0.));
#3798=DIRECTION('center_axis',(0.,0.706957380091336,0.707256150722208));
#3799=DIRECTION('ref_axis',(0.,-0.707256150722208,0.706957380091336));
#3800=DIRECTION('',(0.,-0.707256150722208,0.706957380091336));
#3801=DIRECTION('center_axis',(1.,0.,0.));
#3802=DIRECTION('ref_axis',(0.,1.,0.));
#4458=CARTESIAN_POINT('',(0.,0.,0.));
#4459=CARTESIAN_POINT('Origin',(-40.,0.,-3.02305319600895));
#4460=CARTESIAN_POINT('',(-38.5,1.83697019872103E-16,-2.77305319600895));
#4461=CARTESIAN_POINT('Origin',(-40.,0.,-2.77305319600895));
#4462=CARTESIAN_POINT('',(-38.,-2.44929359829471E-16,-3.27305319600895));
#4463=CARTESIAN_POINT('',(-38.25,-2.14313189850787E-16,-3.02305319600895));
#4464=CARTESIAN_POINT('Origin',(-40.,0.,-3.27305319600895));
#4465=CARTESIAN_POINT('Origin',(0.,0.,-3.27305319600895));
#4466=CARTESIAN_POINT('',(-50.,4.52151022278658,-3.27305319600895));
#4467=CARTESIAN_POINT('',(50.,4.52151022278658,-3.27305319600895));
#4468=CARTESIAN_POINT('',(0.,4.52151022278658,-3.27305319600895));
#4469=CARTESIAN_POINT('',(50.,-4.52151022278658,-3.27305319600895));
#4470=CARTESIAN_POINT('',(50.,-4.52151022278658,-3.27305319600895));
#4471=CARTESIAN_POINT('',(-50.,-4.52151022278658,-3.27305319600895));
#4472=CARTESIAN_POINT('',(0.,-4.52151022278658,-3.27305319600895));
#4473=CARTESIAN_POINT('',(-50.,4.52151022278658,-3.27305319600895));
#4474=CARTESIAN_POINT('',(-18.,-2.4492935982947E-16,-3.27305319600895));
#4475=CARTESIAN_POINT('Origin',(-20.,0.,-3.27305319600895));
#4476=CARTESIAN_POINT('',(22.,-2.44929359829471E-16,-3.27305319600895));
#4477=CARTESIAN_POINT('Origin',(20.,0.,-3.27305319600895));
#4478=CARTESIAN_POINT('',(42.,-2.4492935982947E-16,-3.27305319600895));
#4479=CARTESIAN_POINT('Origin',(40.,0.,-3.27305319600895));
#4480=CARTESIAN_POINT('',(2.,-2.44929359829471E-16,-3.27305319600895));
#4481=CARTESIAN_POINT('Origin',(0.,0.,-3.27305319600895));
#4482=CARTESIAN_POINT('Origin',(-40.,0.,3.27472668609763));
#4483=CARTESIAN_POINT('',(-38.5,1.83697019872103E-16,1.27472668609763));
#4484=CARTESIAN_POINT('Origin',(-40.,0.,1.27472668609763));
#4485=CARTESIAN_POINT('',(-38.5,-1.83697019872103E-16,3.27472668609763));
#4486=CARTESIAN_POINT('Origin',(-20.,0.,-3.02305319600895));
#4487=CARTESIAN_POINT('',(-18.5,1.83697019872103E-16,-2.77305319600895));
#4488=CARTESIAN_POINT('Origin',(-20.,0.,-2.77305319600895));
#4489=CARTESIAN_POINT('',(-18.25,-2.14313189850787E-16,-3.02305319600895));
#4490=CARTESIAN_POINT('Origin',(-20.,0.,3.27472668609763));
#4491=CARTESIAN_POINT('',(-18.5,1.83697019872103E-16,1.27472668609763));
#4492=CARTESIAN_POINT('Origin',(-20.,0.,1.27472668609763));
#4493=CARTESIAN_POINT('',(-18.5,-1.83697019872103E-16,3.27472668609763));
#4494=CARTESIAN_POINT('Origin',(0.,0.,-3.02305319600895));
#4495=CARTESIAN_POINT('',(1.5,1.83697019872103E-16,-2.77305319600895));
#4496=CARTESIAN_POINT('Origin',(0.,0.,-2.77305319600895));
#4497=CARTESIAN_POINT('',(1.75,-2.14313189850787E-16,-3.02305319600895));
#4498=CARTESIAN_POINT('Origin',(0.,0.,3.27472668609763));
#4499=CARTESIAN_POINT('',(1.5,1.83697019872103E-16,1.27472668609763));
#4500=CARTESIAN_POINT('Origin',(0.,0.,1.27472668609763));
#4501=CARTESIAN_POINT('',(1.5,-1.83697019872103E-16,3.27472668609763));
#4502=CARTESIAN_POINT('Origin',(20.,0.,-3.02305319600895));
#4503=CARTESIAN_POINT('',(21.5,1.83697019872103E-16,-2.77305319600895));
#4504=CARTESIAN_POINT('Origin',(20.,0.,-2.77305319600895));
#4505=CARTESIAN_POINT('',(21.75,-2.14313189850787E-16,-3.02305319600895));
#4506=CARTESIAN_POINT('Origin',(20.,0.,3.27472668609763));
#4507=CARTESIAN_POINT('',(21.5,1.83697019872103E-16,1.27472668609763));
#4508=CARTESIAN_POINT('Origin',(20.,0.,1.27472668609763));
#4509=CARTESIAN_POINT('',(21.5,-1.83697019872103E-16,3.27472668609763));
#4510=CARTESIAN_POINT('Origin',(40.,0.,-3.02305319600895));
#4511=CARTESIAN_POINT('',(41.5,1.83697019872103E-16,-2.77305319600895));
#4512=CARTESIAN_POINT('Origin',(40.,0.,-2.77305319600895));
#4513=CARTESIAN_POINT('',(41.75,-2.14313189850787E-16,-3.02305319600895));
#4514=CARTESIAN_POINT('Origin',(40.,0.,3.27472668609763));
#4515=CARTESIAN_POINT('',(41.5,1.83697019872103E-16,1.27472668609763));
#4516=CARTESIAN_POINT('Origin',(40.,0.,1.27472668609763));
#4517=CARTESIAN_POINT('',(41.5,-1.83697019872103E-16,3.27472668609763));
#4518=CARTESIAN_POINT('Origin',(0.,0.,3.27472668609763));
#4519=CARTESIAN_POINT('',(3.,3.67394039744206E-16,3.27472668609763));
#4520=CARTESIAN_POINT('Origin',(0.,0.,3.27472668609763));
#4521=CARTESIAN_POINT('',(3.,3.67394039744206E-16,1.27472668609763));
#4522=CARTESIAN_POINT('',(3.,-3.67394039744206E-16,3.27472668609763));
#4523=CARTESIAN_POINT('Origin',(0.,0.,1.27472668609763));
#4524=CARTESIAN_POINT('Origin',(0.,0.,1.27472668609763));
#4525=CARTESIAN_POINT('Origin',(20.,0.,3.27472668609763));
#4526=CARTESIAN_POINT('',(23.,3.67394039744206E-16,3.27472668609763));
#4527=CARTESIAN_POINT('Origin',(20.,0.,3.27472668609763));
#4528=CARTESIAN_POINT('',(23.,3.67394039744206E-16,1.27472668609763));
#4529=CARTESIAN_POINT('',(23.,-3.67394039744206E-16,3.27472668609763));
#4530=CARTESIAN_POINT('Origin',(20.,0.,1.27472668609763));
#4531=CARTESIAN_POINT('Origin',(20.,0.,1.27472668609763));
#4532=CARTESIAN_POINT('Origin',(-20.,0.,3.27472668609763));
#4533=CARTESIAN_POINT('',(-17.,3.67394039744206E-16,3.27472668609763));
#4534=CARTESIAN_POINT('Origin',(-20.,0.,3.27472668609763));
#4535=CARTESIAN_POINT('',(-17.,3.67394039744206E-16,1.27472668609763));
#4536=CARTESIAN_POINT('',(-17.,-3.67394039744206E-16,3.27472668609763));
#4537=CARTESIAN_POINT('Origin',(-20.,0.,1.27472668609763));
#4538=CARTESIAN_POINT('Origin',(-20.,0.,1.27472668609763));
#4539=CARTESIAN_POINT('Origin',(40.,0.,3.27472668609763));
#4540=CARTESIAN_POINT('',(43.,3.67394039744206E-16,3.27472668609763));
#4541=CARTESIAN_POINT('Origin',(40.,0.,3.27472668609763));
#4542=CARTESIAN_POINT('',(43.,3.67394039744206E-16,1.27472668609763));
#4543=CARTESIAN_POINT('',(43.,-3.67394039744206E-16,3.27472668609763));
#4544=CARTESIAN_POINT('Origin',(40.,0.,1.27472668609763));
#4545=CARTESIAN_POINT('Origin',(40.,0.,1.27472668609763));
#4546=CARTESIAN_POINT('Origin',(-40.,0.,3.27472668609763));
#4547=CARTESIAN_POINT('',(-37.,3.67394039744206E-16,3.27472668609763));
#4548=CARTESIAN_POINT('Origin',(-40.,0.,3.27472668609763));
#4549=CARTESIAN_POINT('',(-37.,3.67394039744206E-16,1.27472668609763));
#4550=CARTESIAN_POINT('',(-37.,-3.67394039744206E-16,3.27472668609763));
#4551=CARTESIAN_POINT('Origin',(-40.,0.,1.27472668609763));
#4552=CARTESIAN_POINT('Origin',(-40.,0.,1.27472668609763));
#4553=CARTESIAN_POINT('Origin',(0.,-4.52151022278658,1.494186706068));
#4554=CARTESIAN_POINT('',(50.,-4.52151022278658,2.73932600723025));
#4555=CARTESIAN_POINT('',(-50.,-4.52151022278658,2.73932600723025));
#4556=CARTESIAN_POINT('',(0.,-4.52151022278658,2.73932600723025));
#4557=CARTESIAN_POINT('',(-50.,-4.52151022278658,1.494186706068));
#4558=CARTESIAN_POINT('',(-50.,-4.52151022278658,3.27472668609763));
#4559=CARTESIAN_POINT('',(50.,-4.52151022278658,1.494186706068));
#4560=CARTESIAN_POINT('',(0.,-4.52151022278658,1.494186706068));
#4561=CARTESIAN_POINT('',(50.,-4.52151022278658,3.27472668609763));
#4562=CARTESIAN_POINT('Origin',(0.,-4.49107020104243,0.747511725556171));
#4563=CARTESIAN_POINT('',(-50.,-4.52151022278657,0.000836745044343612));
#4564=CARTESIAN_POINT('Origin',(-50.,-4.49107020104243,0.747511725556171));
#4565=CARTESIAN_POINT('',(50.,-4.52151022278657,0.000836745044343612));
#4566=CARTESIAN_POINT('',(0.,-4.52151022278657,0.000836745044343579));
#4567=CARTESIAN_POINT('Origin',(50.,-4.49107020104243,0.747511725556171));
#4568=CARTESIAN_POINT('Origin',(0.,-4.52151022278658,-3.27305319600895));
#4569=CARTESIAN_POINT('',(-50.,-4.52151022278658,3.27472668609763));
#4570=CARTESIAN_POINT('',(50.,-4.52151022278658,3.27472668609763));
#4571=CARTESIAN_POINT('Origin',(0.,-4.52151022278658,2.73932600723025));
#4572=CARTESIAN_POINT('',(-50.,-3.98588327568422,3.27472668609763));
#4573=CARTESIAN_POINT('',(50.,-3.98588327568422,3.27472668609763));
#4574=CARTESIAN_POINT('',(0.,-3.98588327568422,3.27472668609763));
#4575=CARTESIAN_POINT('',(-50.,-4.52151022278658,2.73932600723025));
#4576=CARTESIAN_POINT('',(50.,-4.52151022278658,2.73932600723025));
#4577=CARTESIAN_POINT('Origin',(-50.,2.26075511139329,0.000836745044343612));
#4578=CARTESIAN_POINT('',(-50.,3.98588327568422,3.27472668609763));
#4579=CARTESIAN_POINT('',(-50.,4.52151022278658,2.73932600723025));
#4580=CARTESIAN_POINT('',(-50.,4.52151022278658,2.73932600723025));
#4581=CARTESIAN_POINT('',(-50.,4.52151022278658,1.494186706068));
#4582=CARTESIAN_POINT('',(-50.,4.52151022278658,3.27472668609763));
#4583=CARTESIAN_POINT('',(-50.,4.52151022278657,0.000836745044343612));
#4584=CARTESIAN_POINT('Origin',(-50.,4.49107020104243,0.747511725556171));
#4585=CARTESIAN_POINT('',(-50.,4.52151022278658,3.27472668609763));
#4586=CARTESIAN_POINT('',(-50.,0.,3.27472668609763));
#4587=CARTESIAN_POINT('Origin',(0.,4.52151022278658,1.494186706068));
#4588=CARTESIAN_POINT('',(50.,4.52151022278658,2.73932600723025));
#4589=CARTESIAN_POINT('',(0.,4.52151022278658,2.73932600723025));
#4590=CARTESIAN_POINT('',(50.,4.52151022278658,1.494186706068));
#4591=CARTESIAN_POINT('',(50.,4.52151022278658,3.27472668609763));
#4592=CARTESIAN_POINT('',(0.,4.52151022278658,1.494186706068));
#4593=CARTESIAN_POINT('Origin',(0.,4.49107020104243,0.747511725556171));
#4594=CARTESIAN_POINT('',(50.,4.52151022278657,0.000836745044343612));
#4595=CARTESIAN_POINT('Origin',(50.,4.49107020104243,0.747511725556171));
#4596=CARTESIAN_POINT('',(0.,4.52151022278657,0.000836745044343579));
#4597=CARTESIAN_POINT('Origin',(0.,4.52151022278658,-3.27305319600895));
#4598=CARTESIAN_POINT('',(50.,4.52151022278658,3.27472668609763));
#4599=CARTESIAN_POINT('Origin',(0.,3.98588327568422,3.27472668609763));
#4600=CARTESIAN_POINT('',(50.,3.98588327568422,3.27472668609763));
#4601=CARTESIAN_POINT('',(50.,0.,3.27472668609763));
#4602=CARTESIAN_POINT('',(0.,3.98588327568422,3.27472668609763));
#4603=CARTESIAN_POINT('Origin',(0.,4.52151022278658,2.73932600723025));
#4604=CARTESIAN_POINT('',(50.,4.52151022278658,2.73932600723025));
#4605=CARTESIAN_POINT('Origin',(50.,2.26075511139329,0.000836745044343612));
#4976=UNCERTAINTY_MEASURE_WITH_UNIT(LENGTH_MEASURE(0.01),#4995,
'DISTANCE_ACCURACY_VALUE',
'Maximum model space distance between geometric entities at asserted c
onnectivities');
#4982=UNCERTAINTY_MEASURE_WITH_UNIT(LENGTH_MEASURE(0.01),#4995,
'DISTANCE_ACCURACY_VALUE',
'Maximum model space distance between geometric entities at asserted c
onnectivities');
#4988=(
GEOMETRIC_REPRESENTATION_CONTEXT(3)
GLOBAL_UNCERTAINTY_ASSIGNED_CONTEXT((#4976))
GLOBAL_UNIT_ASSIGNED_CONTEXT((#4995,#4997,#4998))
REPRESENTATION_CONTEXT('','3D')
);
#4994=(
GEOMETRIC_REPRESENTATION_CONTEXT(3)
GLOBAL_UNCERTAINTY_ASSIGNED_CONTEXT((#4982))
GLOBAL_UNIT_ASSIGNED_CONTEXT((#4995,#4997,#4998))
REPRESENTATION_CONTEXT('','3D')
);
#4995=(
LENGTH_UNIT()
NAMED_UNIT(*)
SI_UNIT(.MILLI.,.METRE.)
);
#4997=(
NAMED_UNIT(*)
PLANE_ANGLE_UNIT()
SI_UNIT($,.RADIAN.)
);
#4998=(
NAMED_UNIT(*)
SI_UNIT($,.STERADIAN.)
SOLID_ANGLE_UNIT()
);
#5004=SHAPE_DEFINITION_REPRESENTATION(#5015,#5036);
#5015=PRODUCT_DEFINITION_SHAPE('',$,#5048);
#5036=SHAPE_REPRESENTATION('',(#3141),#4988);
#5042=PRODUCT_DEFINITION_CONTEXT('part definition',#5077,'design');
#5048=PRODUCT_DEFINITION('Rail','Rail',#5059,#5042);
#5059=PRODUCT_DEFINITION_FORMATION('',$,#5084);
#5077=APPLICATION_CONTEXT(
'Core Data for Automotive Mechanical Design Process');
#5078=PRODUCT_CONTEXT('part definition',#5077,'mechanical');
#5084=PRODUCT('Rail','Rail',$,(#5078));
#5092=PRESENTATION_STYLE_ASSIGNMENT((#5097));
#5097=SURFACE_STYLE_USAGE(.BOTH.,#5102);
#5102=SURFACE_SIDE_STYLE('',(#5107));
#5107=SURFACE_STYLE_FILL_AREA(#5112);
#5112=FILL_AREA_STYLE('Opaque(211,211,211)',(#5117));
#5117=FILL_AREA_STYLE_COLOUR('Opaque(211,211,211)',#5122);
#5122=COLOUR_RGB('Opaque(211,211,211)', 0.72549020, 0.75294118, 0.79215686);
ENDSEC;
END-ISO-10303-21;
